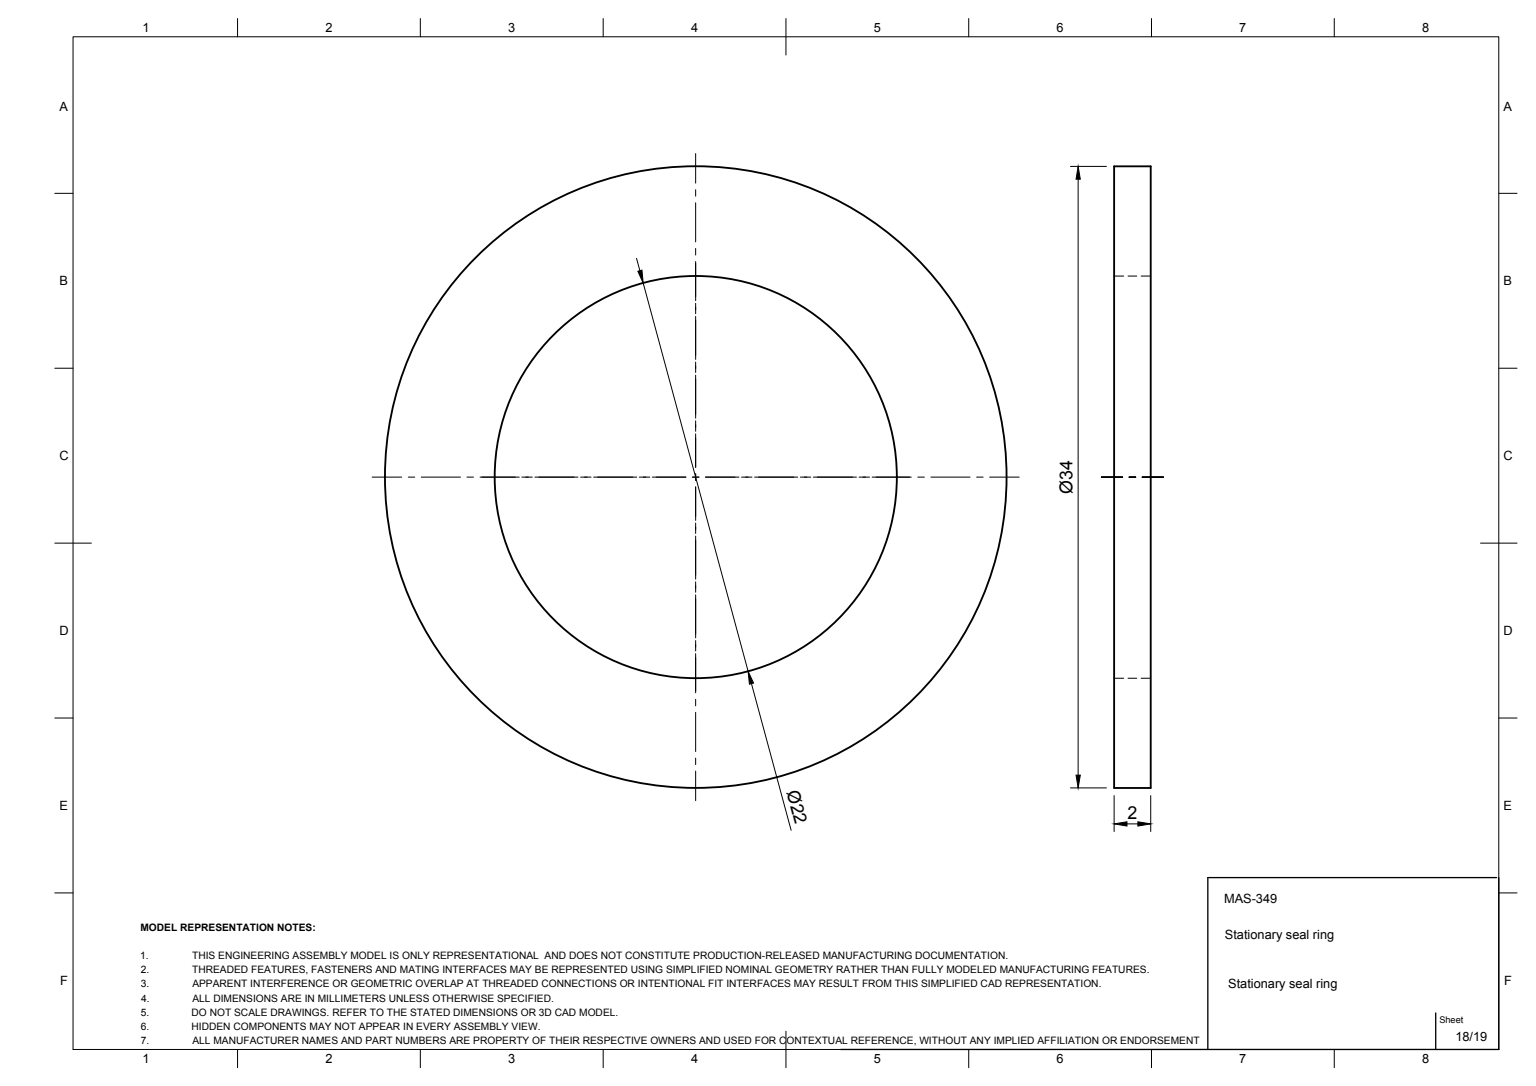
ISO-10303-21;
HEADER;
/* Generated by software containing ST-Developer
 * from STEP Tools, Inc. (www.steptools.com) 
 */

FILE_DESCRIPTION(
/* description */ ('Independent two-stage semi-open centrifugal-pump CAD. Shared impeller
s, open-machinable return casings, removable diaphragms, bronze wear/j
ournal rings, volume-preserving seal instances, retained keyed shaft, 
opposed mechanical face rings and partly threaded tie hardware. Native
 shaft rotation. Geometric topology/clearance only; flow/head/efficien
cy, pressure, cavitation, balance, preload, face loading and secondary
 seal fits/bonds, material/thermal/tolerance selection and life unassi
gned. External drive, coupling, anchors and piping bolts omitted.'),
/* implementation_level */ '2;1');

FILE_NAME(
/* name */ 'Stationary seal ring.step',
/* time_stamp */ '2026-11-08T18:06:32-08:00',
/* author */ (''),
/* organization */ (''),
/* preprocessor_version */ 'ST-DEVELOPER v20.2',
/* originating_system */ 'Autodesk Translation Framework v15.17.0.0',
/* authorisation */ '');

FILE_SCHEMA (('AUTOMOTIVE_DESIGN { 1 0 10303 214 3 1 1 }'));
ENDSEC;

DATA;
#10=MECHANICAL_DESIGN_GEOMETRIC_PRESENTATION_REPRESENTATION('',(#408),#16687);
#370=SHAPE_REPRESENTATION_RELATIONSHIP('SRR','None',#16779,#389);
#389=ADVANCED_BREP_SHAPE_REPRESENTATION('',(#427),#16683);
#408=STYLED_ITEM('',(#16878),#427);
#427=MANIFOLD_SOLID_BREP('Body1',#6127);
#547=FACE_BOUND('',#1454,.T.);
#548=FACE_BOUND('',#1456,.T.);
#667=PLANE('',#6896);
#668=PLANE('',#6897);
#988=FACE_OUTER_BOUND('',#1451,.T.);
#989=FACE_OUTER_BOUND('',#1452,.T.);
#990=FACE_OUTER_BOUND('',#1453,.T.);
#991=FACE_OUTER_BOUND('',#1455,.T.);
#1451=EDGE_LOOP('',(#5353,#5354,#5355,#5356));
#1452=EDGE_LOOP('',(#5357,#5358,#5359,#5360));
#1453=EDGE_LOOP('',(#5361));
#1454=EDGE_LOOP('',(#5362));
#1455=EDGE_LOOP('',(#5363));
#1456=EDGE_LOOP('',(#5364));
#1824=LINE('',#15222,#2193);
#1825=LINE('',#15228,#2194);
#2193=VECTOR('',#8412,1.1);
#2194=VECTOR('',#8419,1.7);
#2478=CIRCLE('',#6891,1.1);
#2479=CIRCLE('',#6892,1.1);
#2480=CIRCLE('',#6894,1.7);
#2481=CIRCLE('',#6895,1.7);
#2985=VERTEX_POINT('',#15219);
#2986=VERTEX_POINT('',#15221);
#2987=VERTEX_POINT('',#15225);
#2988=VERTEX_POINT('',#15227);
#3786=EDGE_CURVE('',#2985,#2985,#2478,.T.);
#3787=EDGE_CURVE('',#2985,#2986,#1824,.T.);
#3788=EDGE_CURVE('',#2986,#2986,#2479,.T.);
#3789=EDGE_CURVE('',#2987,#2987,#2480,.T.);
#3790=EDGE_CURVE('',#2987,#2988,#1825,.T.);
#3791=EDGE_CURVE('',#2988,#2988,#2481,.T.);
#5353=ORIENTED_EDGE('',*,*,#3786,.F.);
#5354=ORIENTED_EDGE('',*,*,#3787,.T.);
#5355=ORIENTED_EDGE('',*,*,#3788,.T.);
#5356=ORIENTED_EDGE('',*,*,#3787,.F.);
#5357=ORIENTED_EDGE('',*,*,#3789,.F.);
#5358=ORIENTED_EDGE('',*,*,#3790,.T.);
#5359=ORIENTED_EDGE('',*,*,#3791,.T.);
#5360=ORIENTED_EDGE('',*,*,#3790,.F.);
#5361=ORIENTED_EDGE('',*,*,#3789,.T.);
#5362=ORIENTED_EDGE('',*,*,#3786,.T.);
#5363=ORIENTED_EDGE('',*,*,#3791,.F.);
#5364=ORIENTED_EDGE('',*,*,#3788,.F.);
#5742=CYLINDRICAL_SURFACE('',#6890,1.1);
#5743=CYLINDRICAL_SURFACE('',#6893,1.7);
#6067=ADVANCED_FACE('',(#988),#5742,.F.);
#6068=ADVANCED_FACE('',(#989),#5743,.T.);
#6069=ADVANCED_FACE('',(#990,#547),#667,.T.);
#6070=ADVANCED_FACE('',(#991,#548),#668,.F.);
#6127=CLOSED_SHELL('',(#6067,#6068,#6069,#6070));
#6889=AXIS2_PLACEMENT_3D('',#15217,#8406,#8407);
#6890=AXIS2_PLACEMENT_3D('',#15218,#8408,#8409);
#6891=AXIS2_PLACEMENT_3D('',#15220,#8410,#8411);
#6892=AXIS2_PLACEMENT_3D('',#15223,#8413,#8414);
#6893=AXIS2_PLACEMENT_3D('',#15224,#8415,#8416);
#6894=AXIS2_PLACEMENT_3D('',#15226,#8417,#8418);
#6895=AXIS2_PLACEMENT_3D('',#15229,#8420,#8421);
#6896=AXIS2_PLACEMENT_3D('',#15230,#8422,#8423);
#6897=AXIS2_PLACEMENT_3D('',#15231,#8424,#8425);
#8406=DIRECTION('axis',(0.,0.,1.));
#8407=DIRECTION('refdir',(1.,0.,0.));
#8408=DIRECTION('center_axis',(0.,0.,1.));
#8409=DIRECTION('ref_axis',(1.,0.,0.));
#8410=DIRECTION('center_axis',(0.,0.,-1.));
#8411=DIRECTION('ref_axis',(1.,0.,0.));
#8412=DIRECTION('',(0.,0.,-1.));
#8413=DIRECTION('center_axis',(0.,0.,-1.));
#8414=DIRECTION('ref_axis',(1.,0.,0.));
#8415=DIRECTION('center_axis',(0.,0.,1.));
#8416=DIRECTION('ref_axis',(1.,0.,0.));
#8417=DIRECTION('center_axis',(0.,0.,1.));
#8418=DIRECTION('ref_axis',(1.,0.,0.));
#8419=DIRECTION('',(0.,0.,-1.));
#8420=DIRECTION('center_axis',(0.,0.,1.));
#8421=DIRECTION('ref_axis',(1.,0.,0.));
#8422=DIRECTION('center_axis',(0.,0.,1.));
#8423=DIRECTION('ref_axis',(1.,0.,0.));
#8424=DIRECTION('center_axis',(0.,0.,1.));
#8425=DIRECTION('ref_axis',(1.,0.,0.));
#15217=CARTESIAN_POINT('',(0.,0.,0.));
#15218=CARTESIAN_POINT('Origin',(0.,0.,11.4));
#15219=CARTESIAN_POINT('',(-1.1,-1.34711147906209E-16,11.6));
#15220=CARTESIAN_POINT('Origin',(0.,0.,11.6));
#15221=CARTESIAN_POINT('',(-1.1,-1.34711147906209E-16,11.4));
#15222=CARTESIAN_POINT('',(-1.1,-1.34711147906209E-16,11.4));
#15223=CARTESIAN_POINT('Origin',(0.,0.,11.4));
#15224=CARTESIAN_POINT('Origin',(0.,0.,11.4));
#15225=CARTESIAN_POINT('',(-1.7,-2.0818995585505E-16,11.6));
#15226=CARTESIAN_POINT('Origin',(0.,0.,11.6));
#15227=CARTESIAN_POINT('',(-1.7,-2.0818995585505E-16,11.4));
#15228=CARTESIAN_POINT('',(-1.7,-2.0818995585505E-16,11.4));
#15229=CARTESIAN_POINT('Origin',(0.,0.,11.4));
#15230=CARTESIAN_POINT('Origin',(0.,0.,11.6));
#15231=CARTESIAN_POINT('Origin',(0.,0.,11.4));
#16662=UNCERTAINTY_MEASURE_WITH_UNIT(LENGTH_MEASURE(0.001),#16688,
'DISTANCE_ACCURACY_VALUE',
'Maximum model space distance between geometric entities at asserted c
onnectivities');
#16666=UNCERTAINTY_MEASURE_WITH_UNIT(LENGTH_MEASURE(0.001),#16688,
'DISTANCE_ACCURACY_VALUE',
'Maximum model space distance between geometric entities at asserted c
onnectivities');
#16683=(
GEOMETRIC_REPRESENTATION_CONTEXT(3)
GLOBAL_UNCERTAINTY_ASSIGNED_CONTEXT((#16662))
GLOBAL_UNIT_ASSIGNED_CONTEXT((#16688,#16690,#16691))
REPRESENTATION_CONTEXT('','3D')
);
#16687=(
GEOMETRIC_REPRESENTATION_CONTEXT(3)
GLOBAL_UNCERTAINTY_ASSIGNED_CONTEXT((#16666))
GLOBAL_UNIT_ASSIGNED_CONTEXT((#16688,#16690,#16691))
REPRESENTATION_CONTEXT('','3D')
);
#16688=(
LENGTH_UNIT()
NAMED_UNIT(*)
SI_UNIT(.CENTI.,.METRE.)
);
#16690=(
NAMED_UNIT(*)
PLANE_ANGLE_UNIT()
SI_UNIT($,.RADIAN.)
);
#16691=(
NAMED_UNIT(*)
SI_UNIT($,.STERADIAN.)
SOLID_ANGLE_UNIT()
);
#16708=SHAPE_DEFINITION_REPRESENTATION(#16728,#16779);
#16728=PRODUCT_DEFINITION_SHAPE('',$,#16800);
#16779=SHAPE_REPRESENTATION('',(#6889),#16683);
#16783=PRODUCT_DEFINITION_CONTEXT('part definition',#16845,'design');
#16800=PRODUCT_DEFINITION('Stationary seal ring','Stationary seal ring',
#16820,#16783);
#16820=PRODUCT_DEFINITION_FORMATION('',$,#16863);
#16845=APPLICATION_CONTEXT(
'Core Data for Automotive Mechanical Design Process');
#16846=PRODUCT_CONTEXT('part definition',#16845,'mechanical');
#16863=PRODUCT('Stationary seal ring','Stationary seal ring',$,(#16846));
#16878=PRESENTATION_STYLE_ASSIGNMENT((#16893));
#16893=SURFACE_STYLE_USAGE(.BOTH.,#16908);
#16908=SURFACE_SIDE_STYLE('',(#16923));
#16923=SURFACE_STYLE_FILL_AREA(#16938);
#16938=FILL_AREA_STYLE('Face seal charcoal',(#16953));
#16953=FILL_AREA_STYLE_COLOUR('Face seal charcoal',#16968);
#16968=COLOUR_RGB('Face seal charcoal',0.164705882352941,0.184313725490196,
0.211764705882353);
ENDSEC;
END-ISO-10303-21;
